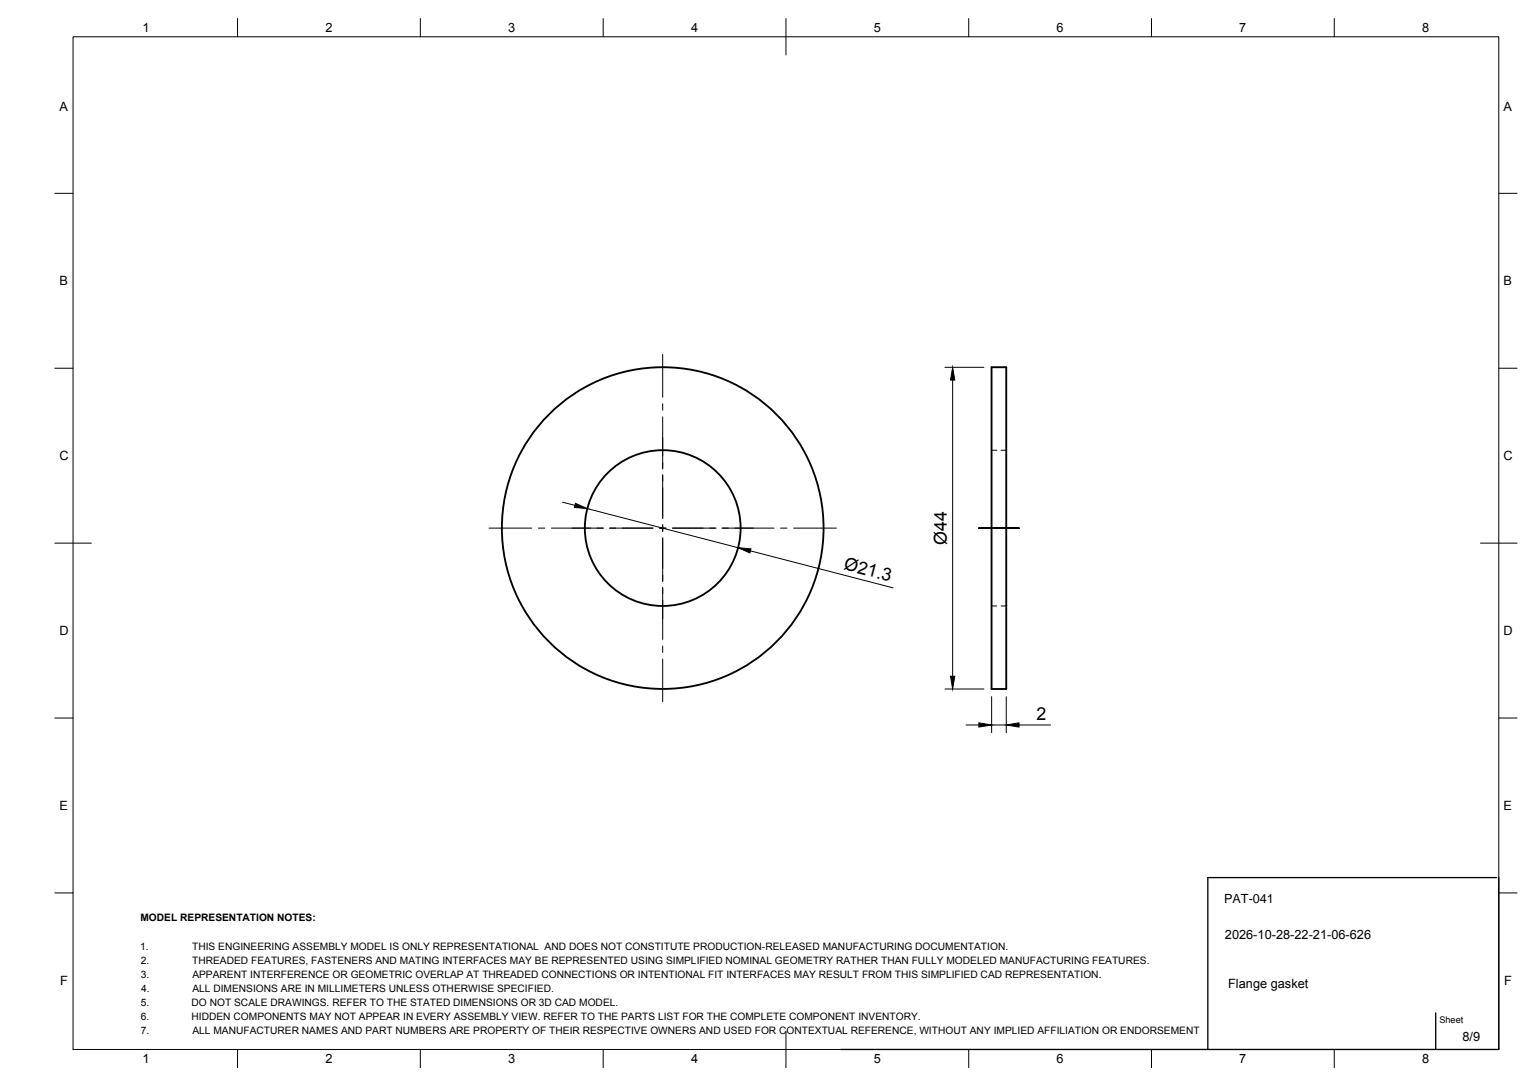
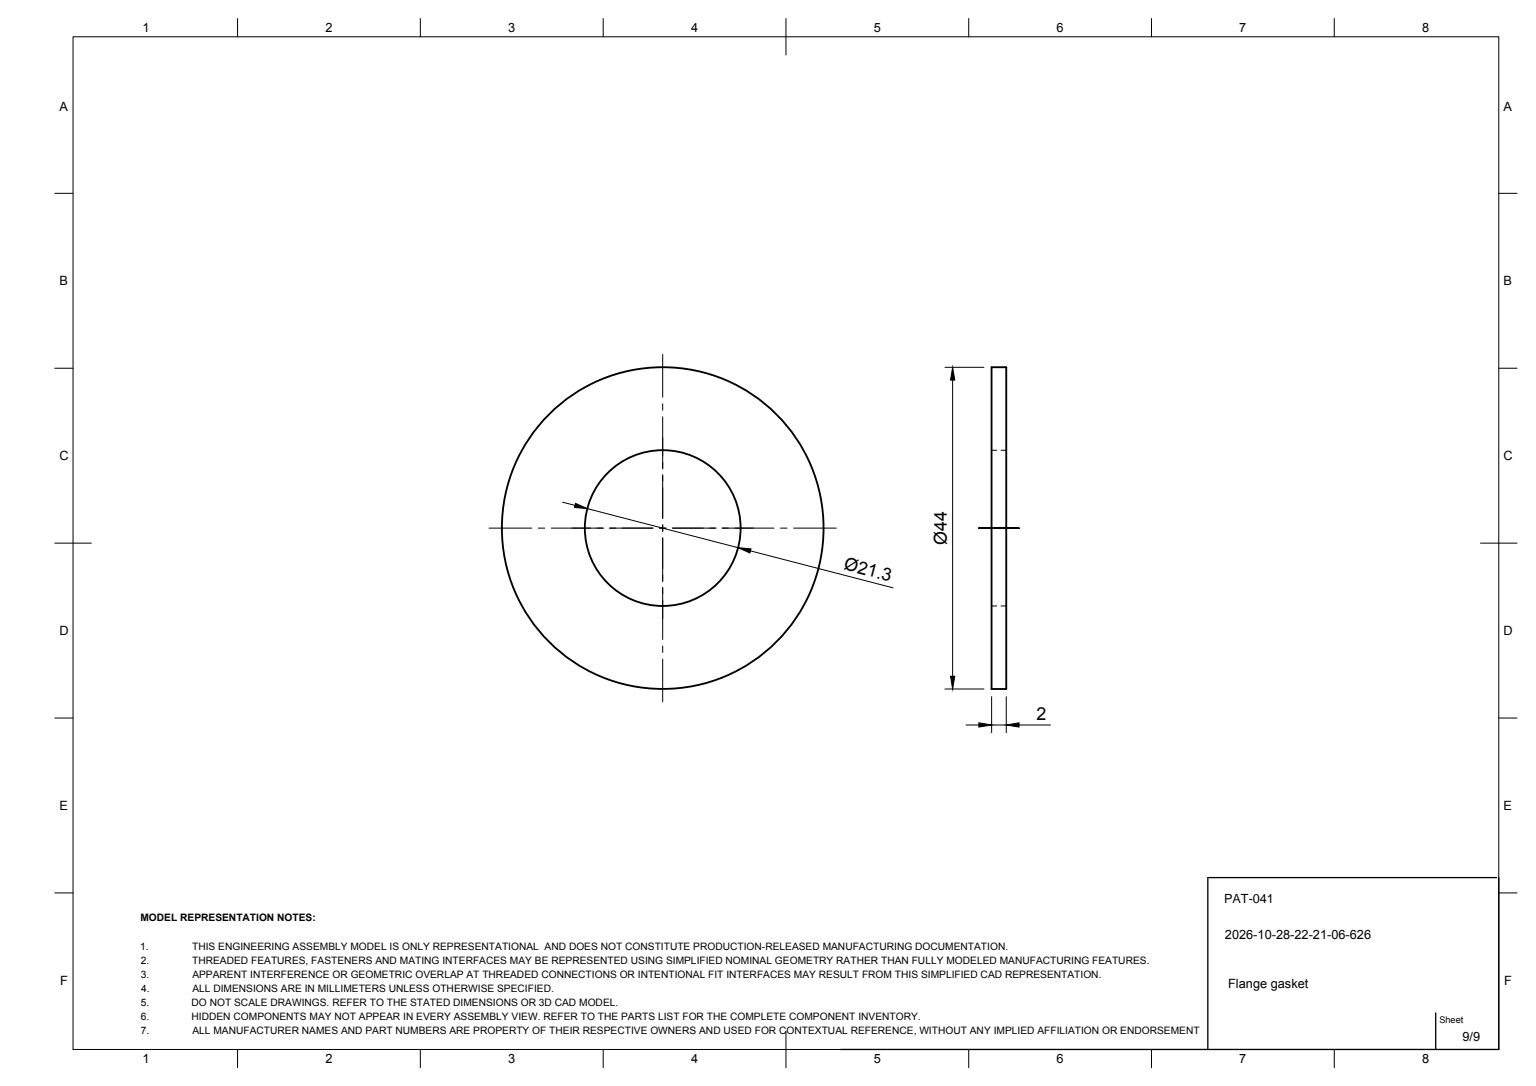
ISO-10303-21;
HEADER;
/* Generated by software containing ST-Developer
 * from STEP Tools, Inc. (www.steptools.com) 
 */

FILE_DESCRIPTION(
/* description */ ('PAT-041'),
/* implementation_level */ '2;1');

FILE_NAME(
/* name */ 'Flange gasket.step',
/* time_stamp */ '2026-10-28T22:21:24-07:00',
/* author */ (''),
/* organization */ (''),
/* preprocessor_version */ 'ST-DEVELOPER v20.2',
/* originating_system */ 'Autodesk Translation Framework v15.17.0.0',
/* authorisation */ '');

FILE_SCHEMA (('AUTOMOTIVE_DESIGN { 1 0 10303 214 3 1 1 }'));
ENDSEC;

DATA;
#10=MECHANICAL_DESIGN_GEOMETRIC_PRESENTATION_REPRESENTATION('',(#214),#2507);
#194=SHAPE_REPRESENTATION_RELATIONSHIP('SRR','None',#2579,#204);
#204=ADVANCED_BREP_SHAPE_REPRESENTATION('',(#224),#2502);
#214=STYLED_ITEM('',(#2708),#224);
#224=MANIFOLD_SOLID_BREP('Body1',#1334);
#271=FACE_BOUND('',#465,.T.);
#272=FACE_BOUND('',#467,.T.);
#290=PLANE('',#1551);
#291=PLANE('',#1552);
#349=FACE_OUTER_BOUND('',#462,.T.);
#350=FACE_OUTER_BOUND('',#463,.T.);
#351=FACE_OUTER_BOUND('',#464,.T.);
#352=FACE_OUTER_BOUND('',#466,.T.);
#462=EDGE_LOOP('',(#1088,#1089,#1090,#1091));
#463=EDGE_LOOP('',(#1092,#1093,#1094,#1095));
#464=EDGE_LOOP('',(#1096));
#465=EDGE_LOOP('',(#1097));
#466=EDGE_LOOP('',(#1098));
#467=EDGE_LOOP('',(#1099));
#532=LINE('',#2262,#588);
#533=LINE('',#2268,#589);
#588=VECTOR('',#1863,1.065);
#589=VECTOR('',#1870,2.2);
#670=CIRCLE('',#1546,1.065);
#671=CIRCLE('',#1547,1.065);
#672=CIRCLE('',#1549,2.2);
#673=CIRCLE('',#1550,2.2);
#742=VERTEX_POINT('',#2259);
#743=VERTEX_POINT('',#2261);
#744=VERTEX_POINT('',#2265);
#745=VERTEX_POINT('',#2267);
#864=EDGE_CURVE('',#742,#742,#670,.T.);
#865=EDGE_CURVE('',#742,#743,#532,.T.);
#866=EDGE_CURVE('',#743,#743,#671,.T.);
#867=EDGE_CURVE('',#744,#744,#672,.T.);
#868=EDGE_CURVE('',#744,#745,#533,.T.);
#869=EDGE_CURVE('',#745,#745,#673,.T.);
#1088=ORIENTED_EDGE('',*,*,#864,.F.);
#1089=ORIENTED_EDGE('',*,*,#865,.T.);
#1090=ORIENTED_EDGE('',*,*,#866,.T.);
#1091=ORIENTED_EDGE('',*,*,#865,.F.);
#1092=ORIENTED_EDGE('',*,*,#867,.F.);
#1093=ORIENTED_EDGE('',*,*,#868,.T.);
#1094=ORIENTED_EDGE('',*,*,#869,.T.);
#1095=ORIENTED_EDGE('',*,*,#868,.F.);
#1096=ORIENTED_EDGE('',*,*,#867,.T.);
#1097=ORIENTED_EDGE('',*,*,#864,.T.);
#1098=ORIENTED_EDGE('',*,*,#869,.F.);
#1099=ORIENTED_EDGE('',*,*,#866,.F.);
#1250=CYLINDRICAL_SURFACE('',#1545,1.065);
#1251=CYLINDRICAL_SURFACE('',#1548,2.2);
#1294=ADVANCED_FACE('',(#349),#1250,.F.);
#1295=ADVANCED_FACE('',(#350),#1251,.T.);
#1296=ADVANCED_FACE('',(#351,#271),#290,.T.);
#1297=ADVANCED_FACE('',(#352,#272),#291,.F.);
#1334=CLOSED_SHELL('',(#1294,#1295,#1296,#1297));
#1544=AXIS2_PLACEMENT_3D('',#2257,#1857,#1858);
#1545=AXIS2_PLACEMENT_3D('',#2258,#1859,#1860);
#1546=AXIS2_PLACEMENT_3D('',#2260,#1861,#1862);
#1547=AXIS2_PLACEMENT_3D('',#2263,#1864,#1865);
#1548=AXIS2_PLACEMENT_3D('',#2264,#1866,#1867);
#1549=AXIS2_PLACEMENT_3D('',#2266,#1868,#1869);
#1550=AXIS2_PLACEMENT_3D('',#2269,#1871,#1872);
#1551=AXIS2_PLACEMENT_3D('',#2270,#1873,#1874);
#1552=AXIS2_PLACEMENT_3D('',#2271,#1875,#1876);
#1857=DIRECTION('axis',(0.,0.,1.));
#1858=DIRECTION('refdir',(1.,0.,0.));
#1859=DIRECTION('center_axis',(1.,0.,0.));
#1860=DIRECTION('ref_axis',(0.,0.,-1.));
#1861=DIRECTION('center_axis',(-1.,0.,0.));
#1862=DIRECTION('ref_axis',(0.,0.,-1.));
#1863=DIRECTION('',(-1.,0.,0.));
#1864=DIRECTION('center_axis',(-1.,0.,0.));
#1865=DIRECTION('ref_axis',(0.,0.,-1.));
#1866=DIRECTION('center_axis',(1.,0.,0.));
#1867=DIRECTION('ref_axis',(0.,0.,-1.));
#1868=DIRECTION('center_axis',(1.,0.,0.));
#1869=DIRECTION('ref_axis',(0.,0.,-1.));
#1870=DIRECTION('',(-1.,0.,0.));
#1871=DIRECTION('center_axis',(1.,0.,0.));
#1872=DIRECTION('ref_axis',(0.,0.,-1.));
#1873=DIRECTION('center_axis',(1.,0.,0.));
#1874=DIRECTION('ref_axis',(0.,0.,-1.));
#1875=DIRECTION('center_axis',(1.,0.,0.));
#1876=DIRECTION('ref_axis',(0.,0.,-1.));
#2257=CARTESIAN_POINT('',(0.,0.,0.));
#2258=CARTESIAN_POINT('Origin',(-10.2,0.,0.));
#2259=CARTESIAN_POINT('',(-10.,-1.30424884109193E-16,1.065));
#2260=CARTESIAN_POINT('Origin',(-10.,0.,0.));
#2261=CARTESIAN_POINT('',(-10.2,-1.30424884109193E-16,1.065));
#2262=CARTESIAN_POINT('',(-10.2,-1.30424884109193E-16,1.065));
#2263=CARTESIAN_POINT('Origin',(-10.2,0.,0.));
#2264=CARTESIAN_POINT('Origin',(-10.2,0.,0.));
#2265=CARTESIAN_POINT('',(-10.,-2.69422295812418E-16,2.2));
#2266=CARTESIAN_POINT('Origin',(-10.,0.,0.));
#2267=CARTESIAN_POINT('',(-10.2,-2.69422295812418E-16,2.2));
#2268=CARTESIAN_POINT('',(-10.2,-2.69422295812418E-16,2.2));
#2269=CARTESIAN_POINT('Origin',(-10.2,0.,0.));
#2270=CARTESIAN_POINT('Origin',(-10.,0.,0.));
#2271=CARTESIAN_POINT('Origin',(-10.2,0.,0.));
#2490=UNCERTAINTY_MEASURE_WITH_UNIT(LENGTH_MEASURE(0.001),#2508,
'DISTANCE_ACCURACY_VALUE',
'Maximum model space distance between geometric entities at asserted c
onnectivities');
#2495=UNCERTAINTY_MEASURE_WITH_UNIT(LENGTH_MEASURE(0.001),#2508,
'DISTANCE_ACCURACY_VALUE',
'Maximum model space distance between geometric entities at asserted c
onnectivities');
#2502=(
GEOMETRIC_REPRESENTATION_CONTEXT(3)
GLOBAL_UNCERTAINTY_ASSIGNED_CONTEXT((#2490))
GLOBAL_UNIT_ASSIGNED_CONTEXT((#2508,#2510,#2511))
REPRESENTATION_CONTEXT('','3D')
);
#2507=(
GEOMETRIC_REPRESENTATION_CONTEXT(3)
GLOBAL_UNCERTAINTY_ASSIGNED_CONTEXT((#2495))
GLOBAL_UNIT_ASSIGNED_CONTEXT((#2508,#2510,#2511))
REPRESENTATION_CONTEXT('','3D')
);
#2508=(
LENGTH_UNIT()
NAMED_UNIT(*)
SI_UNIT(.CENTI.,.METRE.)
);
#2510=(
NAMED_UNIT(*)
PLANE_ANGLE_UNIT()
SI_UNIT($,.RADIAN.)
);
#2511=(
NAMED_UNIT(*)
SI_UNIT($,.STERADIAN.)
SOLID_ANGLE_UNIT()
);
#2518=SHAPE_DEFINITION_REPRESENTATION(#2529,#2579);
#2529=PRODUCT_DEFINITION_SHAPE('',$,#2591);
#2579=SHAPE_REPRESENTATION('',(#1544),#2502);
#2584=PRODUCT_DEFINITION_CONTEXT('part definition',#2619,'design');
#2591=PRODUCT_DEFINITION('Flange gasket','Flange gasket',#2602,
#2584);
#2602=PRODUCT_DEFINITION_FORMATION('',$,#2627);
#2619=APPLICATION_CONTEXT(
'Core Data for Automotive Mechanical Design Process');
#2620=PRODUCT_CONTEXT('part definition',#2619,'mechanical');
#2627=PRODUCT('Flange gasket','Flange gasket',
'Flange gasket',(#2620));
#2702=COLOUR_RGB('Off White',0.89,0.88,0.83);
#2703=FILL_AREA_STYLE_COLOUR('',#2702);
#2704=FILL_AREA_STYLE('',(#2703));
#2705=SURFACE_STYLE_FILL_AREA(#2704);
#2706=SURFACE_SIDE_STYLE('',(#2705));
#2707=SURFACE_STYLE_USAGE(.BOTH.,#2706);
#2708=PRESENTATION_STYLE_ASSIGNMENT((#2707));
ENDSEC;
END-ISO-10303-21;
